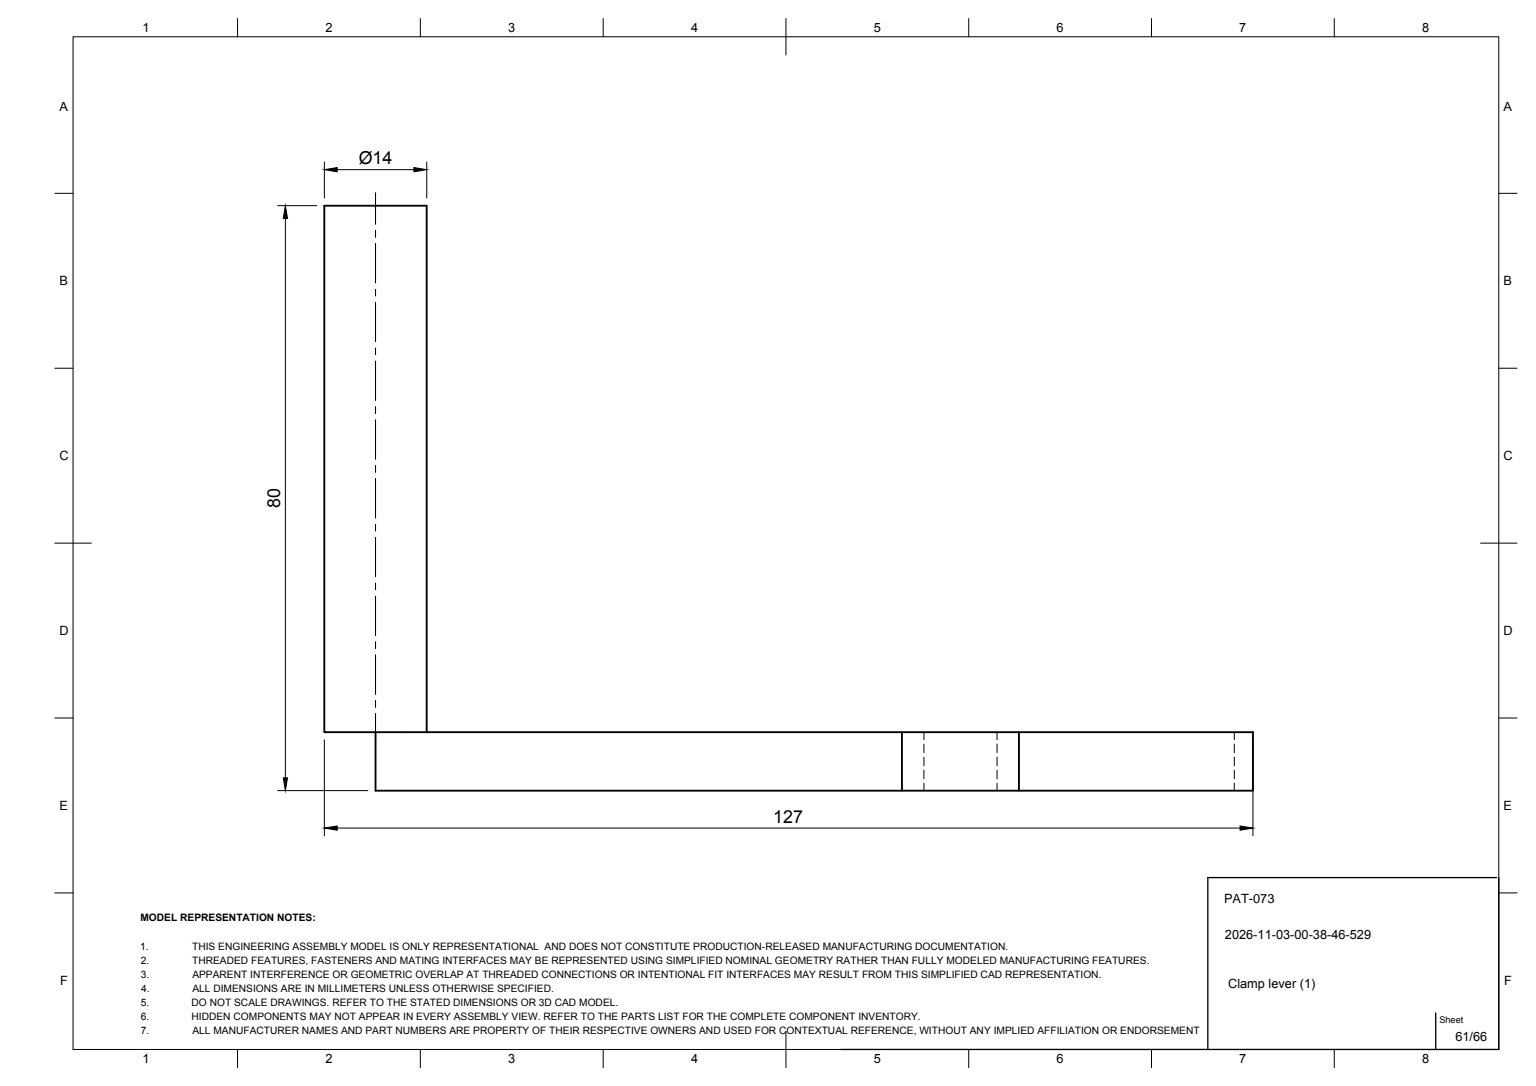
ISO-10303-21;
HEADER;
/* Generated by software containing ST-Developer
 * from STEP Tools, Inc. (www.steptools.com) 
 */

FILE_DESCRIPTION(
/* description */ ('Manual piston pump'),
/* implementation_level */ '2;1');

FILE_NAME(
/* name */ 'Clamp lever (1).step',
/* time_stamp */ '2026-11-02T16:54:23-08:00',
/* author */ (''),
/* organization */ (''),
/* preprocessor_version */ 'ST-DEVELOPER v20.2',
/* originating_system */ 'Autodesk Translation Framework v15.17.0.0',
/* authorisation */ '');

FILE_SCHEMA (('AUTOMOTIVE_DESIGN { 1 0 10303 214 3 1 1 }'));
ENDSEC;

DATA;
#10=MECHANICAL_DESIGN_GEOMETRIC_PRESENTATION_REPRESENTATION('',(#752,#753),#19043);
#618=SHAPE_REPRESENTATION_RELATIONSHIP('SRR','None',#19368,#681);
#681=ADVANCED_BREP_SHAPE_REPRESENTATION('',(#820,#821),#19035);
#752=STYLED_ITEM('',(#19665),#820);
#753=STYLED_ITEM('',(#19665),#821);
#820=MANIFOLD_SOLID_BREP('Body1',#9540);
#821=MANIFOLD_SOLID_BREP('Body2',#9541);
#1033=FACE_BOUND('',#2591,.T.);
#1034=FACE_BOUND('',#2597,.T.);
#1272=CYLINDRICAL_SURFACE('',#11355,0.255000000000001);
#1273=CYLINDRICAL_SURFACE('',#11363,0.5);
#1274=CYLINDRICAL_SURFACE('',#11365,1.);
#1275=CYLINDRICAL_SURFACE('',#11367,1.);
#1276=CYLINDRICAL_SURFACE('',#11376,0.699999999999999);
#1808=FACE_OUTER_BOUND('',#2589,.T.);
#1809=FACE_OUTER_BOUND('',#2590,.T.);
#1810=FACE_OUTER_BOUND('',#2592,.T.);
#1811=FACE_OUTER_BOUND('',#2593,.T.);
#1812=FACE_OUTER_BOUND('',#2594,.T.);
#1813=FACE_OUTER_BOUND('',#2595,.T.);
#1814=FACE_OUTER_BOUND('',#2596,.T.);
#1815=FACE_OUTER_BOUND('',#2598,.T.);
#1816=FACE_OUTER_BOUND('',#2599,.T.);
#1817=FACE_OUTER_BOUND('',#2600,.T.);
#1818=FACE_OUTER_BOUND('',#2601,.T.);
#1819=FACE_OUTER_BOUND('',#2602,.T.);
#1820=FACE_OUTER_BOUND('',#2603,.T.);
#1821=FACE_OUTER_BOUND('',#2604,.T.);
#1822=FACE_OUTER_BOUND('',#2605,.T.);
#1823=FACE_OUTER_BOUND('',#2606,.T.);
#2589=EDGE_LOOP('',(#8351,#8352,#8353,#8354));
#2590=EDGE_LOOP('',(#8355,#8356,#8357,#8358,#8359,#8360,#8361,#8362,#8363,
#8364));
#2591=EDGE_LOOP('',(#8365));
#2592=EDGE_LOOP('',(#8366,#8367,#8368,#8369));
#2593=EDGE_LOOP('',(#8370,#8371,#8372,#8373));
#2594=EDGE_LOOP('',(#8374,#8375,#8376,#8377));
#2595=EDGE_LOOP('',(#8378,#8379,#8380,#8381));
#2596=EDGE_LOOP('',(#8382,#8383,#8384,#8385,#8386,#8387,#8388,#8389,#8390,
#8391));
#2597=EDGE_LOOP('',(#8392));
#2598=EDGE_LOOP('',(#8393,#8394,#8395,#8396));
#2599=EDGE_LOOP('',(#8397,#8398,#8399,#8400));
#2600=EDGE_LOOP('',(#8401,#8402,#8403,#8404));
#2601=EDGE_LOOP('',(#8405,#8406,#8407,#8408));
#2602=EDGE_LOOP('',(#8409,#8410,#8411,#8412));
#2603=EDGE_LOOP('',(#8413,#8414,#8415,#8416));
#2604=EDGE_LOOP('',(#8417,#8418,#8419,#8420));
#2605=EDGE_LOOP('',(#8421));
#2606=EDGE_LOOP('',(#8422));
#3104=CIRCLE('',#11356,0.255000000000001);
#3105=CIRCLE('',#11357,0.255000000000001);
#3106=CIRCLE('',#11359,1.);
#3107=CIRCLE('',#11360,1.);
#3108=CIRCLE('',#11361,0.5);
#3109=CIRCLE('',#11364,0.5);
#3110=CIRCLE('',#11366,1.);
#3111=CIRCLE('',#11368,1.);
#3112=CIRCLE('',#11377,0.699999999999999);
#3113=CIRCLE('',#11378,0.699999999999999);
#3683=LINE('',#18626,#4287);
#3684=LINE('',#18629,#4288);
#3685=LINE('',#18632,#4289);
#3686=LINE('',#18634,#4290);
#3687=LINE('',#18638,#4291);
#3688=LINE('',#18640,#4292);
#3689=LINE('',#18642,#4293);
#3690=LINE('',#18646,#4294);
#3691=LINE('',#18647,#4295);
#3692=LINE('',#18652,#4296);
#3693=LINE('',#18653,#4297);
#3694=LINE('',#18656,#4298);
#3695=LINE('',#18660,#4299);
#3696=LINE('',#18663,#4300);
#3697=LINE('',#18666,#4301);
#3698=LINE('',#18668,#4302);
#3699=LINE('',#18672,#4303);
#3700=LINE('',#18673,#4304);
#3701=LINE('',#18675,#4305);
#3702=LINE('',#18677,#4306);
#3703=LINE('',#18678,#4307);
#3704=LINE('',#18679,#4308);
#3705=LINE('',#18682,#4309);
#3706=LINE('',#18684,#4310);
#3707=LINE('',#18686,#4311);
#3708=LINE('',#18693,#4312);
#4287=VECTOR('',#14259,1.);
#4288=VECTOR('',#14262,1.);
#4289=VECTOR('',#14265,1.);
#4290=VECTOR('',#14266,1.);
#4291=VECTOR('',#14269,1.);
#4292=VECTOR('',#14270,1.);
#4293=VECTOR('',#14271,1.);
#4294=VECTOR('',#14274,1.);
#4295=VECTOR('',#14275,1.);
#4296=VECTOR('',#14280,1.);
#4297=VECTOR('',#14281,1.);
#4298=VECTOR('',#14284,0.5);
#4299=VECTOR('',#14289,1.);
#4300=VECTOR('',#14292,1.);
#4301=VECTOR('',#14295,1.);
#4302=VECTOR('',#14296,1.);
#4303=VECTOR('',#14301,1.);
#4304=VECTOR('',#14302,1.);
#4305=VECTOR('',#14303,1.);
#4306=VECTOR('',#14304,1.);
#4307=VECTOR('',#14305,1.);
#4308=VECTOR('',#14306,1.);
#4309=VECTOR('',#14311,1.);
#4310=VECTOR('',#14314,1.);
#4311=VECTOR('',#14317,1.);
#4312=VECTOR('',#14326,0.699999999999999);
#5050=VERTEX_POINT('',#18622);
#5051=VERTEX_POINT('',#18623);
#5052=VERTEX_POINT('',#18625);
#5053=VERTEX_POINT('',#18627);
#5054=VERTEX_POINT('',#18631);
#5055=VERTEX_POINT('',#18633);
#5056=VERTEX_POINT('',#18635);
#5057=VERTEX_POINT('',#18637);
#5058=VERTEX_POINT('',#18639);
#5059=VERTEX_POINT('',#18641);
#5060=VERTEX_POINT('',#18643);
#5061=VERTEX_POINT('',#18645);
#5062=VERTEX_POINT('',#18648);
#5063=VERTEX_POINT('',#18651);
#5064=VERTEX_POINT('',#18655);
#5065=VERTEX_POINT('',#18659);
#5066=VERTEX_POINT('',#18661);
#5067=VERTEX_POINT('',#18665);
#5068=VERTEX_POINT('',#18667);
#5069=VERTEX_POINT('',#18671);
#5070=VERTEX_POINT('',#18674);
#5071=VERTEX_POINT('',#18676);
#5072=VERTEX_POINT('',#18690);
#5073=VERTEX_POINT('',#18692);
#6162=EDGE_CURVE('',#5050,#5051,#3104,.T.);
#6163=EDGE_CURVE('',#5052,#5050,#3683,.T.);
#6164=EDGE_CURVE('',#5053,#5052,#3105,.T.);
#6165=EDGE_CURVE('',#5051,#5053,#3684,.T.);
#6166=EDGE_CURVE('',#5054,#5052,#3685,.T.);
#6167=EDGE_CURVE('',#5055,#5054,#3686,.T.);
#6168=EDGE_CURVE('',#5056,#5055,#3106,.T.);
#6169=EDGE_CURVE('',#5057,#5056,#3687,.T.);
#6170=EDGE_CURVE('',#5058,#5057,#3688,.T.);
#6171=EDGE_CURVE('',#5059,#5058,#3689,.T.);
#6172=EDGE_CURVE('',#5060,#5059,#3107,.T.);
#6173=EDGE_CURVE('',#5061,#5060,#3690,.T.);
#6174=EDGE_CURVE('',#5053,#5061,#3691,.T.);
#6175=EDGE_CURVE('',#5062,#5062,#3108,.T.);
#6176=EDGE_CURVE('',#5063,#5050,#3692,.T.);
#6177=EDGE_CURVE('',#5054,#5063,#3693,.T.);
#6178=EDGE_CURVE('',#5062,#5064,#3694,.T.);
#6179=EDGE_CURVE('',#5064,#5064,#3109,.T.);
#6180=EDGE_CURVE('',#5065,#5059,#3695,.T.);
#6181=EDGE_CURVE('',#5066,#5065,#3110,.T.);
#6182=EDGE_CURVE('',#5060,#5066,#3696,.T.);
#6183=EDGE_CURVE('',#5056,#5067,#3697,.T.);
#6184=EDGE_CURVE('',#5068,#5055,#3698,.T.);
#6185=EDGE_CURVE('',#5067,#5068,#3111,.T.);
#6186=EDGE_CURVE('',#5051,#5069,#3699,.T.);
#6187=EDGE_CURVE('',#5069,#5066,#3700,.T.);
#6188=EDGE_CURVE('',#5065,#5070,#3701,.T.);
#6189=EDGE_CURVE('',#5070,#5071,#3702,.T.);
#6190=EDGE_CURVE('',#5071,#5067,#3703,.T.);
#6191=EDGE_CURVE('',#5068,#5063,#3704,.T.);
#6192=EDGE_CURVE('',#5061,#5069,#3705,.T.);
#6193=EDGE_CURVE('',#5057,#5071,#3706,.T.);
#6194=EDGE_CURVE('',#5058,#5070,#3707,.T.);
#6195=EDGE_CURVE('',#5072,#5072,#3112,.T.);
#6196=EDGE_CURVE('',#5072,#5073,#3708,.T.);
#6197=EDGE_CURVE('',#5073,#5073,#3113,.T.);
#8351=ORIENTED_EDGE('',*,*,#6162,.F.);
#8352=ORIENTED_EDGE('',*,*,#6163,.F.);
#8353=ORIENTED_EDGE('',*,*,#6164,.F.);
#8354=ORIENTED_EDGE('',*,*,#6165,.F.);
#8355=ORIENTED_EDGE('',*,*,#6164,.T.);
#8356=ORIENTED_EDGE('',*,*,#6166,.F.);
#8357=ORIENTED_EDGE('',*,*,#6167,.F.);
#8358=ORIENTED_EDGE('',*,*,#6168,.F.);
#8359=ORIENTED_EDGE('',*,*,#6169,.F.);
#8360=ORIENTED_EDGE('',*,*,#6170,.F.);
#8361=ORIENTED_EDGE('',*,*,#6171,.F.);
#8362=ORIENTED_EDGE('',*,*,#6172,.F.);
#8363=ORIENTED_EDGE('',*,*,#6173,.F.);
#8364=ORIENTED_EDGE('',*,*,#6174,.F.);
#8365=ORIENTED_EDGE('',*,*,#6175,.T.);
#8366=ORIENTED_EDGE('',*,*,#6163,.T.);
#8367=ORIENTED_EDGE('',*,*,#6176,.F.);
#8368=ORIENTED_EDGE('',*,*,#6177,.F.);
#8369=ORIENTED_EDGE('',*,*,#6166,.T.);
#8370=ORIENTED_EDGE('',*,*,#6175,.F.);
#8371=ORIENTED_EDGE('',*,*,#6178,.T.);
#8372=ORIENTED_EDGE('',*,*,#6179,.F.);
#8373=ORIENTED_EDGE('',*,*,#6178,.F.);
#8374=ORIENTED_EDGE('',*,*,#6180,.F.);
#8375=ORIENTED_EDGE('',*,*,#6181,.F.);
#8376=ORIENTED_EDGE('',*,*,#6182,.F.);
#8377=ORIENTED_EDGE('',*,*,#6172,.T.);
#8378=ORIENTED_EDGE('',*,*,#6183,.F.);
#8379=ORIENTED_EDGE('',*,*,#6168,.T.);
#8380=ORIENTED_EDGE('',*,*,#6184,.F.);
#8381=ORIENTED_EDGE('',*,*,#6185,.F.);
#8382=ORIENTED_EDGE('',*,*,#6162,.T.);
#8383=ORIENTED_EDGE('',*,*,#6186,.T.);
#8384=ORIENTED_EDGE('',*,*,#6187,.T.);
#8385=ORIENTED_EDGE('',*,*,#6181,.T.);
#8386=ORIENTED_EDGE('',*,*,#6188,.T.);
#8387=ORIENTED_EDGE('',*,*,#6189,.T.);
#8388=ORIENTED_EDGE('',*,*,#6190,.T.);
#8389=ORIENTED_EDGE('',*,*,#6185,.T.);
#8390=ORIENTED_EDGE('',*,*,#6191,.T.);
#8391=ORIENTED_EDGE('',*,*,#6176,.T.);
#8392=ORIENTED_EDGE('',*,*,#6179,.T.);
#8393=ORIENTED_EDGE('',*,*,#6184,.T.);
#8394=ORIENTED_EDGE('',*,*,#6167,.T.);
#8395=ORIENTED_EDGE('',*,*,#6177,.T.);
#8396=ORIENTED_EDGE('',*,*,#6191,.F.);
#8397=ORIENTED_EDGE('',*,*,#6182,.T.);
#8398=ORIENTED_EDGE('',*,*,#6187,.F.);
#8399=ORIENTED_EDGE('',*,*,#6192,.F.);
#8400=ORIENTED_EDGE('',*,*,#6173,.T.);
#8401=ORIENTED_EDGE('',*,*,#6183,.T.);
#8402=ORIENTED_EDGE('',*,*,#6190,.F.);
#8403=ORIENTED_EDGE('',*,*,#6193,.F.);
#8404=ORIENTED_EDGE('',*,*,#6169,.T.);
#8405=ORIENTED_EDGE('',*,*,#6170,.T.);
#8406=ORIENTED_EDGE('',*,*,#6193,.T.);
#8407=ORIENTED_EDGE('',*,*,#6189,.F.);
#8408=ORIENTED_EDGE('',*,*,#6194,.F.);
#8409=ORIENTED_EDGE('',*,*,#6180,.T.);
#8410=ORIENTED_EDGE('',*,*,#6171,.T.);
#8411=ORIENTED_EDGE('',*,*,#6194,.T.);
#8412=ORIENTED_EDGE('',*,*,#6188,.F.);
#8413=ORIENTED_EDGE('',*,*,#6165,.T.);
#8414=ORIENTED_EDGE('',*,*,#6174,.T.);
#8415=ORIENTED_EDGE('',*,*,#6192,.T.);
#8416=ORIENTED_EDGE('',*,*,#6186,.F.);
#8417=ORIENTED_EDGE('',*,*,#6195,.F.);
#8418=ORIENTED_EDGE('',*,*,#6196,.T.);
#8419=ORIENTED_EDGE('',*,*,#6197,.T.);
#8420=ORIENTED_EDGE('',*,*,#6196,.F.);
#8421=ORIENTED_EDGE('',*,*,#6195,.T.);
#8422=ORIENTED_EDGE('',*,*,#6197,.F.);
#8861=PLANE('',#11358);
#8862=PLANE('',#11362);
#8863=PLANE('',#11369);
#8864=PLANE('',#11370);
#8865=PLANE('',#11371);
#8866=PLANE('',#11372);
#8867=PLANE('',#11373);
#8868=PLANE('',#11374);
#8869=PLANE('',#11375);
#8870=PLANE('',#11379);
#8871=PLANE('',#11380);
#9413=ADVANCED_FACE('',(#1808),#1272,.F.);
#9414=ADVANCED_FACE('',(#1809,#1033),#8861,.F.);
#9415=ADVANCED_FACE('',(#1810),#8862,.T.);
#9416=ADVANCED_FACE('',(#1811),#1273,.F.);
#9417=ADVANCED_FACE('',(#1812),#1274,.T.);
#9418=ADVANCED_FACE('',(#1813),#1275,.T.);
#9419=ADVANCED_FACE('',(#1814,#1034),#8863,.T.);
#9420=ADVANCED_FACE('',(#1815),#8864,.T.);
#9421=ADVANCED_FACE('',(#1816),#8865,.T.);
#9422=ADVANCED_FACE('',(#1817),#8866,.T.);
#9423=ADVANCED_FACE('',(#1818),#8867,.T.);
#9424=ADVANCED_FACE('',(#1819),#8868,.T.);
#9425=ADVANCED_FACE('',(#1820),#8869,.T.);
#9426=ADVANCED_FACE('',(#1821),#1276,.T.);
#9427=ADVANCED_FACE('',(#1822),#8870,.T.);
#9428=ADVANCED_FACE('',(#1823),#8871,.F.);
#9540=CLOSED_SHELL('',(#9413,#9414,#9415,#9416,#9417,#9418,#9419,#9420,
#9421,#9422,#9423,#9424,#9425));
#9541=CLOSED_SHELL('',(#9426,#9427,#9428));
#11354=AXIS2_PLACEMENT_3D('',#18620,#14253,#14254);
#11355=AXIS2_PLACEMENT_3D('',#18621,#14255,#14256);
#11356=AXIS2_PLACEMENT_3D('',#18624,#14257,#14258);
#11357=AXIS2_PLACEMENT_3D('',#18628,#14260,#14261);
#11358=AXIS2_PLACEMENT_3D('',#18630,#14263,#14264);
#11359=AXIS2_PLACEMENT_3D('',#18636,#14267,#14268);
#11360=AXIS2_PLACEMENT_3D('',#18644,#14272,#14273);
#11361=AXIS2_PLACEMENT_3D('',#18649,#14276,#14277);
#11362=AXIS2_PLACEMENT_3D('',#18650,#14278,#14279);
#11363=AXIS2_PLACEMENT_3D('',#18654,#14282,#14283);
#11364=AXIS2_PLACEMENT_3D('',#18657,#14285,#14286);
#11365=AXIS2_PLACEMENT_3D('',#18658,#14287,#14288);
#11366=AXIS2_PLACEMENT_3D('',#18662,#14290,#14291);
#11367=AXIS2_PLACEMENT_3D('',#18664,#14293,#14294);
#11368=AXIS2_PLACEMENT_3D('',#18669,#14297,#14298);
#11369=AXIS2_PLACEMENT_3D('',#18670,#14299,#14300);
#11370=AXIS2_PLACEMENT_3D('',#18680,#14307,#14308);
#11371=AXIS2_PLACEMENT_3D('',#18681,#14309,#14310);
#11372=AXIS2_PLACEMENT_3D('',#18683,#14312,#14313);
#11373=AXIS2_PLACEMENT_3D('',#18685,#14315,#14316);
#11374=AXIS2_PLACEMENT_3D('',#18687,#14318,#14319);
#11375=AXIS2_PLACEMENT_3D('',#18688,#14320,#14321);
#11376=AXIS2_PLACEMENT_3D('',#18689,#14322,#14323);
#11377=AXIS2_PLACEMENT_3D('',#18691,#14324,#14325);
#11378=AXIS2_PLACEMENT_3D('',#18694,#14327,#14328);
#11379=AXIS2_PLACEMENT_3D('',#18695,#14329,#14330);
#11380=AXIS2_PLACEMENT_3D('',#18696,#14331,#14332);
#14253=DIRECTION('axis',(0.,0.,1.));
#14254=DIRECTION('refdir',(1.,0.,0.));
#14255=DIRECTION('center_axis',(1.,0.,0.));
#14256=DIRECTION('ref_axis',(0.,0.,-1.));
#14257=DIRECTION('center_axis',(-1.,0.,0.));
#14258=DIRECTION('ref_axis',(0.,0.,-1.));
#14259=DIRECTION('',(1.,0.,0.));
#14260=DIRECTION('center_axis',(1.,0.,0.));
#14261=DIRECTION('ref_axis',(0.,0.,-1.));
#14262=DIRECTION('',(-1.,0.,0.));
#14263=DIRECTION('center_axis',(1.,0.,0.));
#14264=DIRECTION('ref_axis',(0.,0.,-1.));
#14265=DIRECTION('',(0.,0.,-1.));
#14266=DIRECTION('',(0.,-1.,0.));
#14267=DIRECTION('center_axis',(1.,0.,0.));
#14268=DIRECTION('ref_axis',(0.,0.,-1.));
#14269=DIRECTION('',(0.,-1.,0.));
#14270=DIRECTION('',(0.,0.,1.));
#14271=DIRECTION('',(0.,1.,0.));
#14272=DIRECTION('center_axis',(1.,0.,0.));
#14273=DIRECTION('ref_axis',(0.,0.,-1.));
#14274=DIRECTION('',(0.,1.,0.));
#14275=DIRECTION('',(0.,0.,-1.));
#14276=DIRECTION('center_axis',(1.,0.,0.));
#14277=DIRECTION('ref_axis',(0.,0.,-1.));
#14278=DIRECTION('center_axis',(0.,-1.,0.));
#14279=DIRECTION('ref_axis',(0.,0.,-1.));
#14280=DIRECTION('',(0.,0.,-1.));
#14281=DIRECTION('',(1.,0.,0.));
#14282=DIRECTION('center_axis',(1.,0.,0.));
#14283=DIRECTION('ref_axis',(0.,0.,-1.));
#14284=DIRECTION('',(1.,0.,0.));
#14285=DIRECTION('center_axis',(-1.,0.,0.));
#14286=DIRECTION('ref_axis',(0.,0.,-1.));
#14287=DIRECTION('center_axis',(1.,0.,0.));
#14288=DIRECTION('ref_axis',(0.,0.,-1.));
#14289=DIRECTION('',(-1.,0.,0.));
#14290=DIRECTION('center_axis',(1.,0.,0.));
#14291=DIRECTION('ref_axis',(0.,0.,-1.));
#14292=DIRECTION('',(1.,0.,0.));
#14293=DIRECTION('center_axis',(1.,0.,0.));
#14294=DIRECTION('ref_axis',(0.,1.22464679914735E-16,1.));
#14295=DIRECTION('',(1.,0.,0.));
#14296=DIRECTION('',(-1.,0.,0.));
#14297=DIRECTION('center_axis',(1.,0.,0.));
#14298=DIRECTION('ref_axis',(0.,0.,-1.));
#14299=DIRECTION('center_axis',(1.,0.,0.));
#14300=DIRECTION('ref_axis',(0.,0.,-1.));
#14301=DIRECTION('',(0.,0.,-1.));
#14302=DIRECTION('',(0.,1.,0.));
#14303=DIRECTION('',(0.,1.,0.));
#14304=DIRECTION('',(0.,0.,1.));
#14305=DIRECTION('',(0.,-1.,0.));
#14306=DIRECTION('',(0.,-1.,0.));
#14307=DIRECTION('center_axis',(0.,0.,1.));
#14308=DIRECTION('ref_axis',(0.,-1.,0.));
#14309=DIRECTION('center_axis',(0.,0.,-1.));
#14310=DIRECTION('ref_axis',(0.,1.,0.));
#14311=DIRECTION('',(1.,0.,0.));
#14312=DIRECTION('center_axis',(0.,0.,1.));
#14313=DIRECTION('ref_axis',(0.,-1.,0.));
#14314=DIRECTION('',(1.,0.,0.));
#14315=DIRECTION('center_axis',(0.,1.,0.));
#14316=DIRECTION('ref_axis',(0.,0.,1.));
#14317=DIRECTION('',(1.,0.,0.));
#14318=DIRECTION('center_axis',(0.,0.,-1.));
#14319=DIRECTION('ref_axis',(0.,1.,0.));
#14320=DIRECTION('center_axis',(0.,-1.,0.));
#14321=DIRECTION('ref_axis',(0.,0.,-1.));
#14322=DIRECTION('center_axis',(1.,0.,0.));
#14323=DIRECTION('ref_axis',(0.,0.,-1.));
#14324=DIRECTION('center_axis',(1.,0.,0.));
#14325=DIRECTION('ref_axis',(0.,0.,-1.));
#14326=DIRECTION('',(-1.,0.,0.));
#14327=DIRECTION('center_axis',(1.,0.,0.));
#14328=DIRECTION('ref_axis',(0.,0.,-1.));
#14329=DIRECTION('center_axis',(1.,0.,0.));
#14330=DIRECTION('ref_axis',(0.,0.,-1.));
#14331=DIRECTION('center_axis',(1.,0.,0.));
#14332=DIRECTION('ref_axis',(0.,0.,-1.));
#18620=CARTESIAN_POINT('',(0.,0.,0.));
#18621=CARTESIAN_POINT('Origin',(-1.5,-8.,10.));
#18622=CARTESIAN_POINT('',(-0.6,-8.,10.255));
#18623=CARTESIAN_POINT('',(-0.6,-8.,9.745));
#18624=CARTESIAN_POINT('Origin',(-0.6,-8.,10.));
#18625=CARTESIAN_POINT('',(-1.4,-8.,10.255));
#18626=CARTESIAN_POINT('',(-1.5,-8.,10.255));
#18627=CARTESIAN_POINT('',(-1.4,-8.,9.745));
#18628=CARTESIAN_POINT('Origin',(-1.4,-8.,10.));
#18629=CARTESIAN_POINT('',(-1.5,-8.,9.745));
#18630=CARTESIAN_POINT('Origin',(-1.4,-2.,10.));
#18631=CARTESIAN_POINT('',(-1.4,-8.,10.6));
#18632=CARTESIAN_POINT('',(-1.4,-8.,10.6));
#18633=CARTESIAN_POINT('',(-1.4,-4.8,10.6));
#18634=CARTESIAN_POINT('',(-1.4,4.,10.6));
#18635=CARTESIAN_POINT('',(-1.4,-3.2,10.6));
#18636=CARTESIAN_POINT('Origin',(-1.4,-4.,10.));
#18637=CARTESIAN_POINT('',(-1.4,4.,10.6));
#18638=CARTESIAN_POINT('',(-1.4,4.,10.6));
#18639=CARTESIAN_POINT('',(-1.4,4.,9.4));
#18640=CARTESIAN_POINT('',(-1.4,4.,9.4));
#18641=CARTESIAN_POINT('',(-1.4,-3.2,9.4));
#18642=CARTESIAN_POINT('',(-1.4,-8.,9.4));
#18643=CARTESIAN_POINT('',(-1.4,-4.8,9.4));
#18644=CARTESIAN_POINT('Origin',(-1.4,-4.,10.));
#18645=CARTESIAN_POINT('',(-1.4,-8.,9.4));
#18646=CARTESIAN_POINT('',(-1.4,-8.,9.4));
#18647=CARTESIAN_POINT('',(-1.4,-8.,10.6));
#18648=CARTESIAN_POINT('',(-1.4,-4.,10.5));
#18649=CARTESIAN_POINT('Origin',(-1.4,-4.,10.));
#18650=CARTESIAN_POINT('Origin',(-1.4,-8.,10.6));
#18651=CARTESIAN_POINT('',(-0.6,-8.,10.6));
#18652=CARTESIAN_POINT('',(-0.6,-8.,10.6));
#18653=CARTESIAN_POINT('',(-1.4,-8.,10.6));
#18654=CARTESIAN_POINT('Origin',(-1.5,-4.,10.));
#18655=CARTESIAN_POINT('',(-0.6,-4.,10.5));
#18656=CARTESIAN_POINT('',(-1.5,-4.,10.5));
#18657=CARTESIAN_POINT('Origin',(-0.6,-4.,10.));
#18658=CARTESIAN_POINT('Origin',(-1.4,-4.,10.));
#18659=CARTESIAN_POINT('',(-0.6,-3.2,9.4));
#18660=CARTESIAN_POINT('',(-1.4,-3.2,9.4));
#18661=CARTESIAN_POINT('',(-0.6,-4.8,9.4));
#18662=CARTESIAN_POINT('Origin',(-0.6,-4.,10.));
#18663=CARTESIAN_POINT('',(-1.4,-4.8,9.4));
#18664=CARTESIAN_POINT('Origin',(-1.4,-4.,10.));
#18665=CARTESIAN_POINT('',(-0.6,-3.2,10.6));
#18666=CARTESIAN_POINT('',(-1.4,-3.2,10.6));
#18667=CARTESIAN_POINT('',(-0.6,-4.8,10.6));
#18668=CARTESIAN_POINT('',(-1.4,-4.8,10.6));
#18669=CARTESIAN_POINT('Origin',(-0.6,-4.,10.));
#18670=CARTESIAN_POINT('Origin',(-0.6,-2.,10.));
#18671=CARTESIAN_POINT('',(-0.6,-8.,9.4));
#18672=CARTESIAN_POINT('',(-0.6,-8.,10.6));
#18673=CARTESIAN_POINT('',(-0.6,-8.,9.4));
#18674=CARTESIAN_POINT('',(-0.6,4.,9.4));
#18675=CARTESIAN_POINT('',(-0.6,-8.,9.4));
#18676=CARTESIAN_POINT('',(-0.6,4.,10.6));
#18677=CARTESIAN_POINT('',(-0.6,4.,9.4));
#18678=CARTESIAN_POINT('',(-0.6,4.,10.6));
#18679=CARTESIAN_POINT('',(-0.6,4.,10.6));
#18680=CARTESIAN_POINT('Origin',(-1.4,4.,10.6));
#18681=CARTESIAN_POINT('Origin',(-1.4,-8.,9.4));
#18682=CARTESIAN_POINT('',(-1.4,-8.,9.4));
#18683=CARTESIAN_POINT('Origin',(-1.4,4.,10.6));
#18684=CARTESIAN_POINT('',(-1.4,4.,10.6));
#18685=CARTESIAN_POINT('Origin',(-1.4,4.,9.4));
#18686=CARTESIAN_POINT('',(-1.4,4.,9.4));
#18687=CARTESIAN_POINT('Origin',(-1.4,-8.,9.4));
#18688=CARTESIAN_POINT('Origin',(-1.4,-8.,10.6));
#18689=CARTESIAN_POINT('Origin',(-0.6,4.,10.));
#18690=CARTESIAN_POINT('',(6.6,4.,10.7));
#18691=CARTESIAN_POINT('Origin',(6.6,4.,10.));
#18692=CARTESIAN_POINT('',(-0.6,4.,10.7));
#18693=CARTESIAN_POINT('',(-0.6,4.,10.7));
#18694=CARTESIAN_POINT('Origin',(-0.6,4.,10.));
#18695=CARTESIAN_POINT('Origin',(6.6,4.,10.));
#18696=CARTESIAN_POINT('Origin',(-0.6,4.,10.));
#18964=UNCERTAINTY_MEASURE_WITH_UNIT(LENGTH_MEASURE(0.001),#19044,
'DISTANCE_ACCURACY_VALUE',
'Maximum model space distance between geometric entities at asserted c
onnectivities');
#18972=UNCERTAINTY_MEASURE_WITH_UNIT(LENGTH_MEASURE(0.001),#19044,
'DISTANCE_ACCURACY_VALUE',
'Maximum model space distance between geometric entities at asserted c
onnectivities');
#19035=(
GEOMETRIC_REPRESENTATION_CONTEXT(3)
GLOBAL_UNCERTAINTY_ASSIGNED_CONTEXT((#18964))
GLOBAL_UNIT_ASSIGNED_CONTEXT((#19044,#19046,#19047))
REPRESENTATION_CONTEXT('','3D')
);
#19043=(
GEOMETRIC_REPRESENTATION_CONTEXT(3)
GLOBAL_UNCERTAINTY_ASSIGNED_CONTEXT((#18972))
GLOBAL_UNIT_ASSIGNED_CONTEXT((#19044,#19046,#19047))
REPRESENTATION_CONTEXT('','3D')
);
#19044=(
LENGTH_UNIT()
NAMED_UNIT(*)
SI_UNIT(.CENTI.,.METRE.)
);
#19046=(
NAMED_UNIT(*)
PLANE_ANGLE_UNIT()
SI_UNIT($,.RADIAN.)
);
#19047=(
NAMED_UNIT(*)
SI_UNIT($,.STERADIAN.)
SOLID_ANGLE_UNIT()
);
#19110=SHAPE_DEFINITION_REPRESENTATION(#19267,#19368);
#19267=PRODUCT_DEFINITION_SHAPE('',$,#19439);
#19368=SHAPE_REPRESENTATION('',(#11354),#19035);
#19376=PRODUCT_DEFINITION_CONTEXT('part definition',#19588,'design');
#19439=PRODUCT_DEFINITION('2026-11-03-00-38-46-529','Clamp lever (1)',#19509,
#19376);
#19509=PRODUCT_DEFINITION_FORMATION('',$,#19652);
#19588=APPLICATION_CONTEXT(
'Core Data for Automotive Mechanical Design Process');
#19589=PRODUCT_CONTEXT('part definition',#19588,'mechanical');
#19652=PRODUCT('2026-11-03-00-38-46-529','Clamp lever (1)',
'Clamp lever',(#19589));
#19665=PRESENTATION_STYLE_ASSIGNMENT((#19671));
#19671=SURFACE_STYLE_USAGE(.BOTH.,#19677);
#19677=SURFACE_SIDE_STYLE('',(#19683));
#19683=SURFACE_STYLE_FILL_AREA(#19689);
#19689=FILL_AREA_STYLE('CAD Library Painted - Light blue',(#19695));
#19695=FILL_AREA_STYLE_COLOUR('CAD Library Painted - Light blue',#19701);
#19701=COLOUR_RGB('CAD Library Painted - Light blue',0.286274509803922,
0.552941176470588,0.780392156862745);
ENDSEC;
END-ISO-10303-21;
